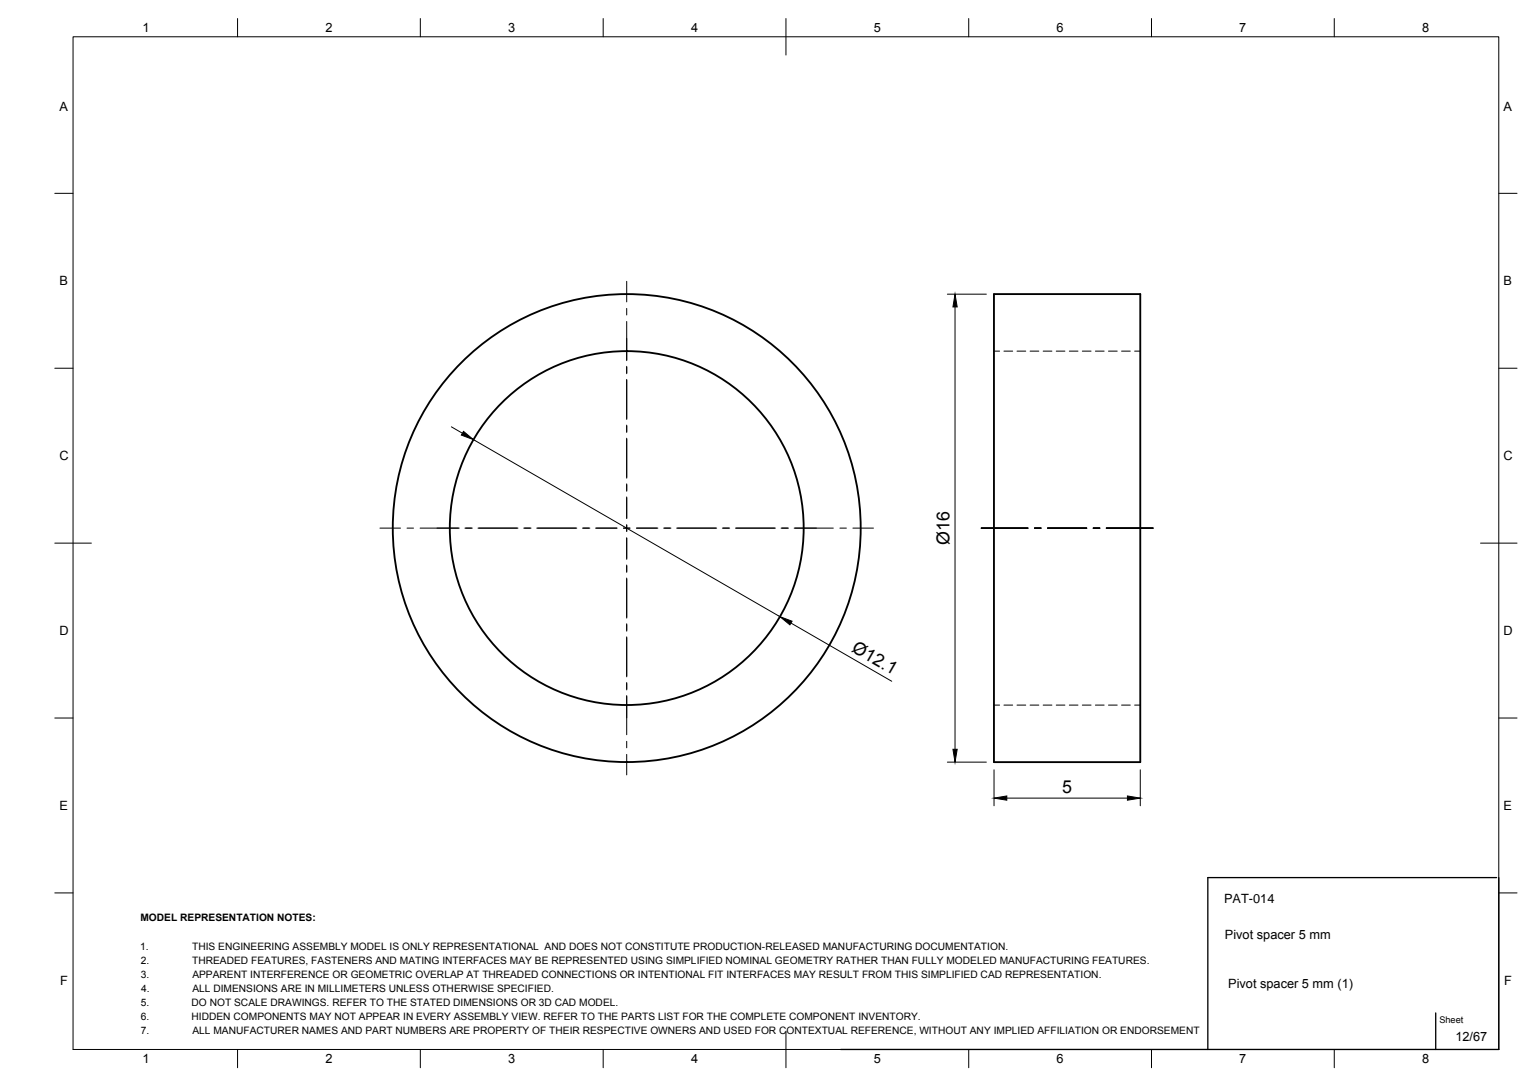
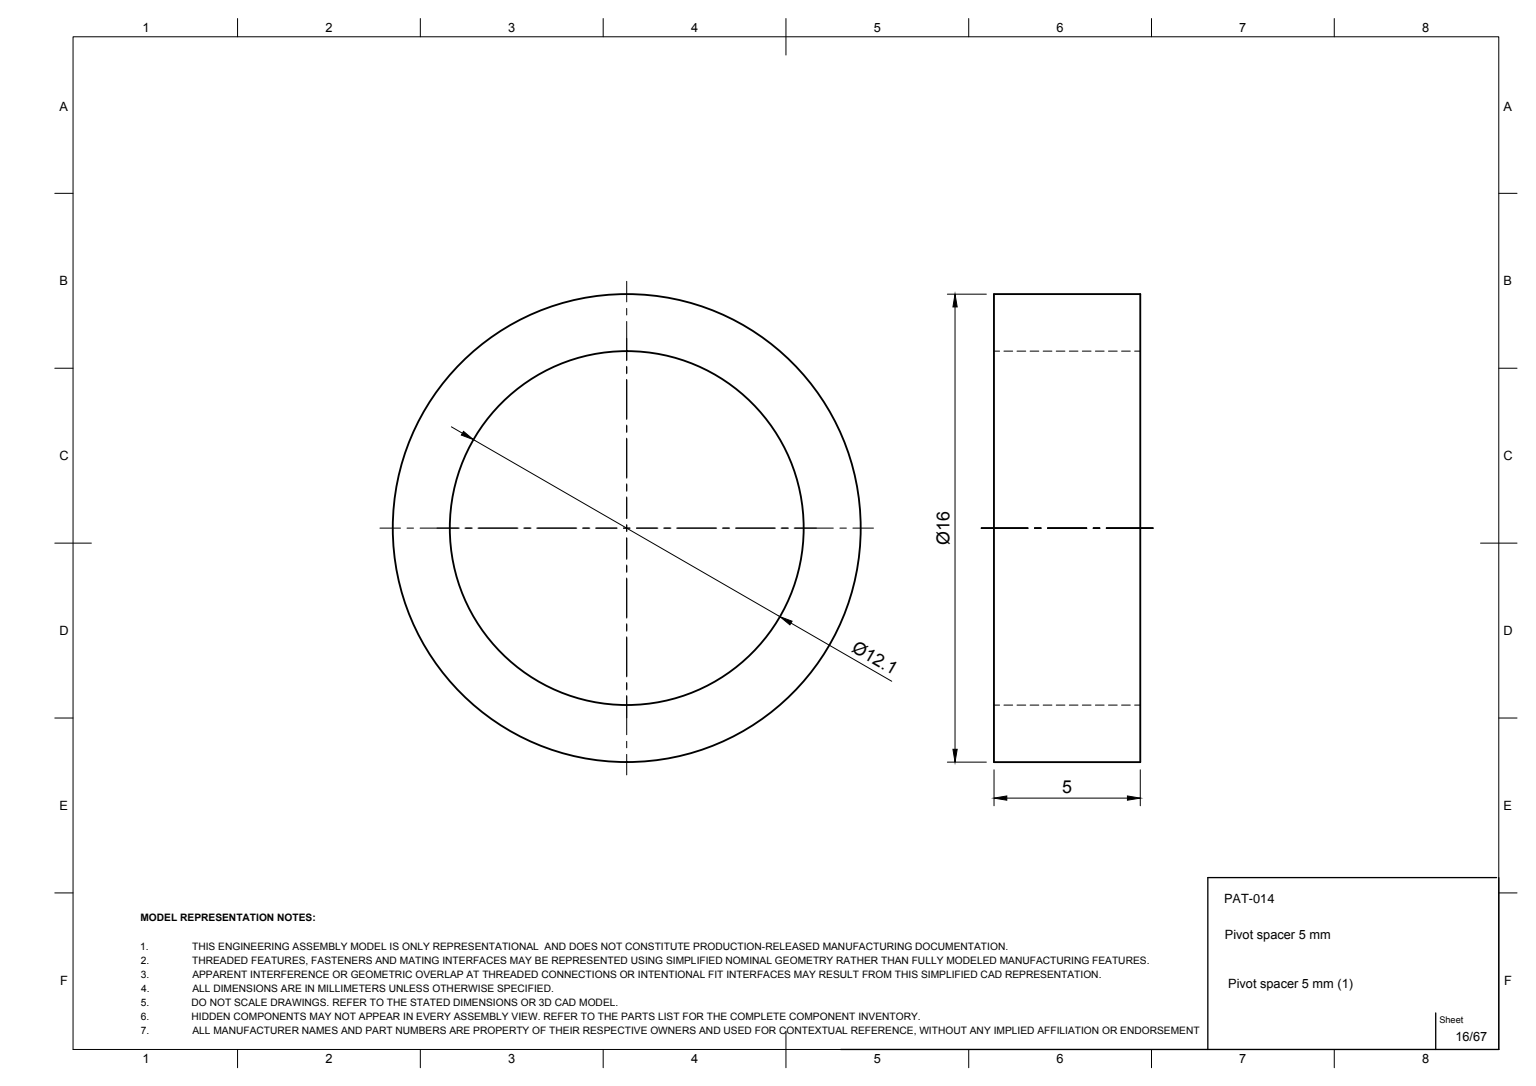
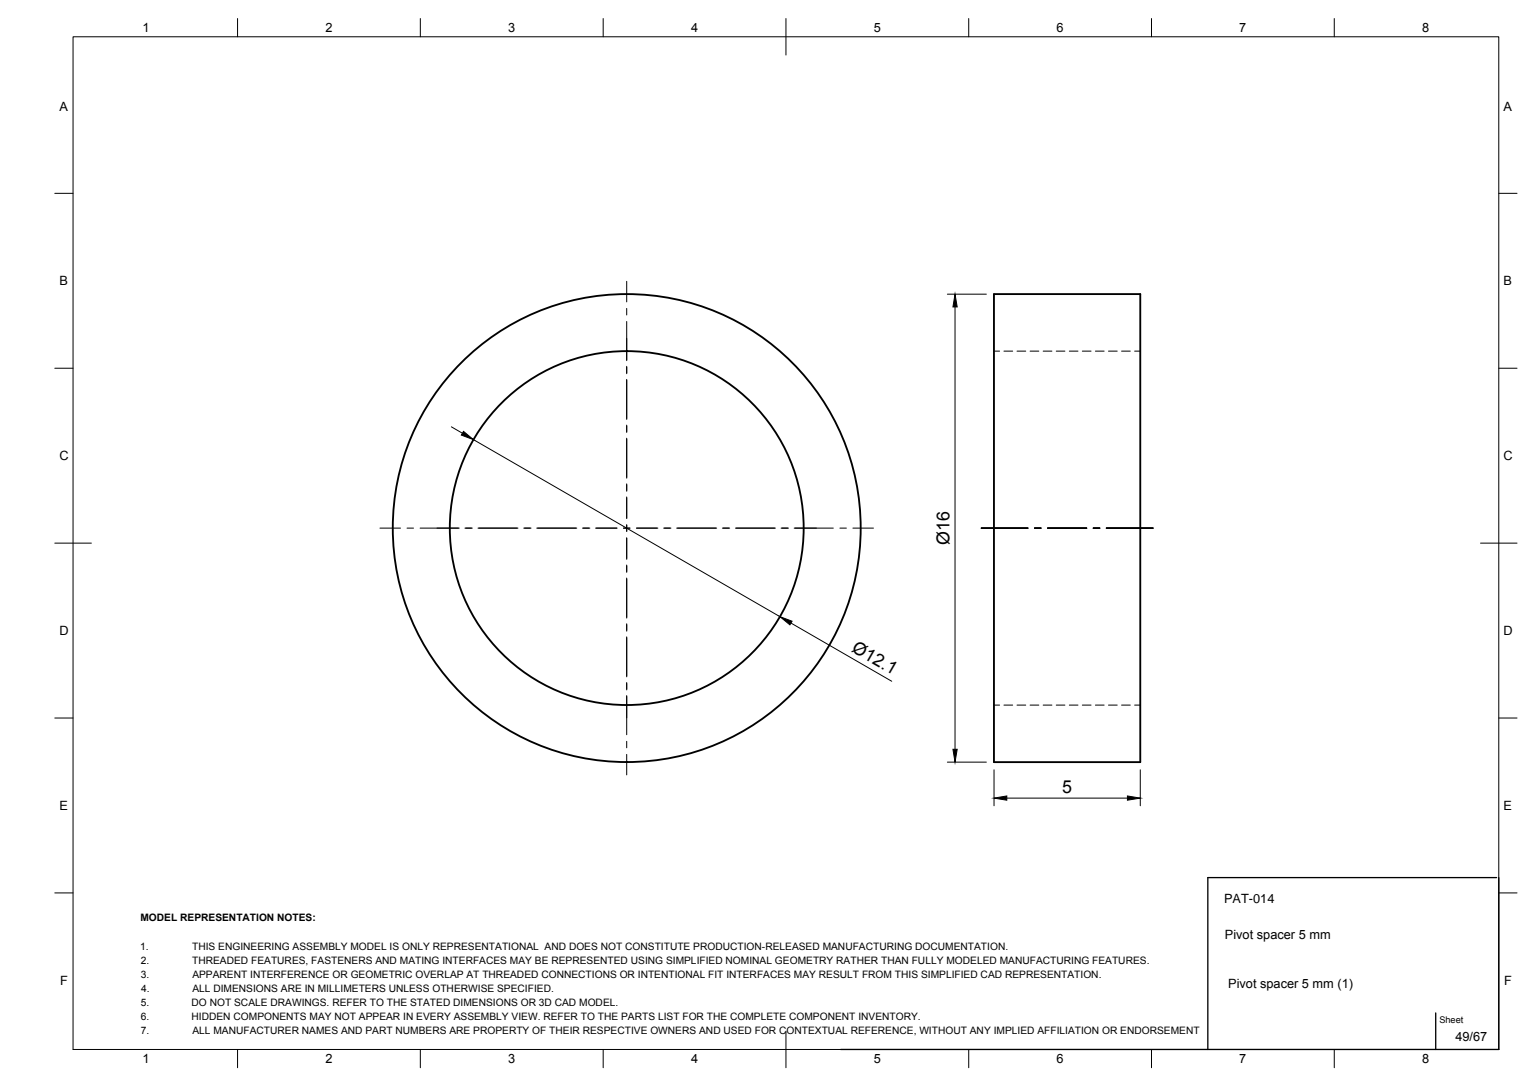
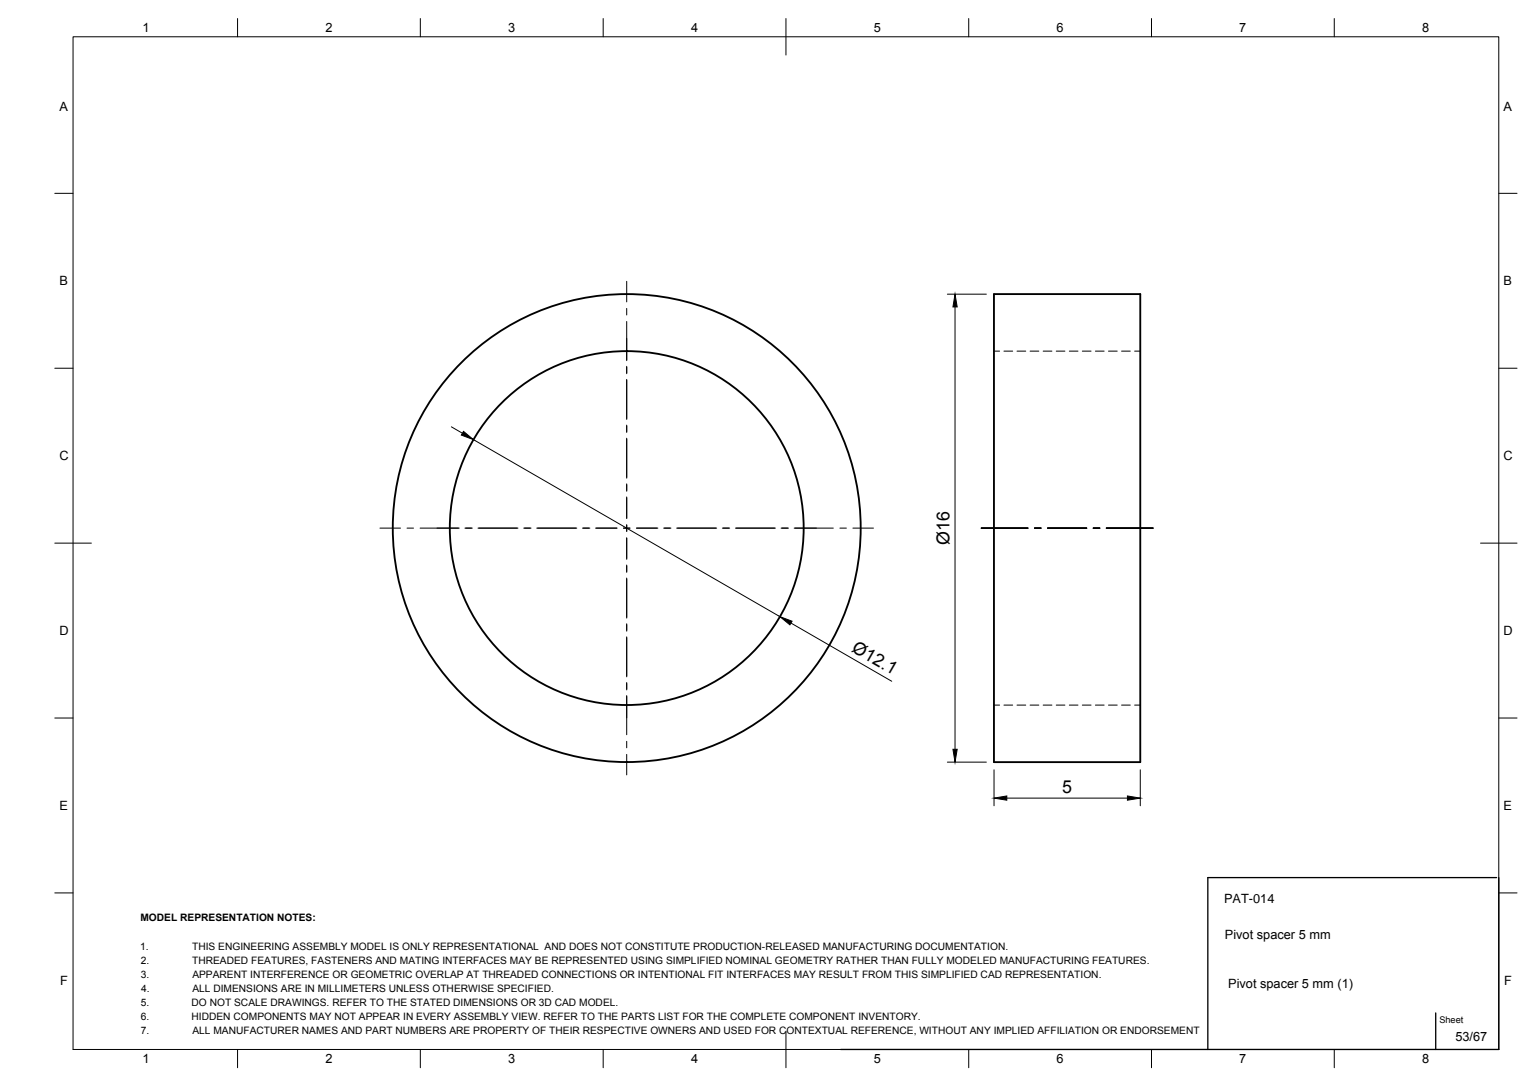
ISO-10303-21;
HEADER;
/* Generated by software containing ST-Developer
 * from STEP Tools, Inc. (www.steptools.com) 
 */

FILE_DESCRIPTION(
/* description */ ('Bin tilter linkage'),
/* implementation_level */ '2;1');

FILE_NAME(
/* name */ 'Pivot spacer 5 mm.step',
/* time_stamp */ '2026-10-28T03:26:24-07:00',
/* author */ (''),
/* organization */ (''),
/* preprocessor_version */ 'ST-DEVELOPER v20.2',
/* originating_system */ 'Autodesk Translation Framework v15.17.0.0',
/* authorisation */ '');

FILE_SCHEMA (('AUTOMOTIVE_DESIGN { 1 0 10303 214 3 1 1 }'));
ENDSEC;

DATA;
#10=MECHANICAL_DESIGN_GEOMETRIC_PRESENTATION_REPRESENTATION('',(#869),#23728);
#657=SHAPE_REPRESENTATION_RELATIONSHIP('SRR','None',#24121,#763);
#763=ADVANCED_BREP_SHAPE_REPRESENTATION('',(#983),#23621);
#869=STYLED_ITEM('',(#24779),#983);
#983=MANIFOLD_SOLID_BREP('Body1',#12399);
#1154=FACE_BOUND('',#2819,.T.);
#1155=FACE_BOUND('',#2821,.T.);
#1537=PLANE('',#13848);
#1538=PLANE('',#13849);
#1972=FACE_OUTER_BOUND('',#2816,.T.);
#1973=FACE_OUTER_BOUND('',#2817,.T.);
#1974=FACE_OUTER_BOUND('',#2818,.T.);
#1975=FACE_OUTER_BOUND('',#2820,.T.);
#2816=EDGE_LOOP('',(#8763,#8764,#8765,#8766));
#2817=EDGE_LOOP('',(#8767,#8768,#8769,#8770));
#2818=EDGE_LOOP('',(#8771));
#2819=EDGE_LOOP('',(#8772));
#2820=EDGE_LOOP('',(#8773));
#2821=EDGE_LOOP('',(#8774));
#3970=LINE('',#20166,#4645);
#3971=LINE('',#20172,#4646);
#4645=VECTOR('',#15931,0.605);
#4646=VECTOR('',#15938,0.8);
#5273=CIRCLE('',#13843,0.605);
#5274=CIRCLE('',#13844,0.605);
#5275=CIRCLE('',#13846,0.8);
#5276=CIRCLE('',#13847,0.8);
#6087=VERTEX_POINT('',#20163);
#6088=VERTEX_POINT('',#20165);
#6089=VERTEX_POINT('',#20169);
#6090=VERTEX_POINT('',#20171);
#7121=EDGE_CURVE('',#6087,#6087,#5273,.T.);
#7122=EDGE_CURVE('',#6087,#6088,#3970,.T.);
#7123=EDGE_CURVE('',#6088,#6088,#5274,.T.);
#7124=EDGE_CURVE('',#6089,#6089,#5275,.T.);
#7125=EDGE_CURVE('',#6089,#6090,#3971,.T.);
#7126=EDGE_CURVE('',#6090,#6090,#5276,.T.);
#8763=ORIENTED_EDGE('',*,*,#7121,.F.);
#8764=ORIENTED_EDGE('',*,*,#7122,.T.);
#8765=ORIENTED_EDGE('',*,*,#7123,.T.);
#8766=ORIENTED_EDGE('',*,*,#7122,.F.);
#8767=ORIENTED_EDGE('',*,*,#7124,.F.);
#8768=ORIENTED_EDGE('',*,*,#7125,.T.);
#8769=ORIENTED_EDGE('',*,*,#7126,.T.);
#8770=ORIENTED_EDGE('',*,*,#7125,.F.);
#8771=ORIENTED_EDGE('',*,*,#7124,.T.);
#8772=ORIENTED_EDGE('',*,*,#7121,.T.);
#8773=ORIENTED_EDGE('',*,*,#7126,.F.);
#8774=ORIENTED_EDGE('',*,*,#7123,.F.);
#11304=CYLINDRICAL_SURFACE('',#13842,0.605);
#11305=CYLINDRICAL_SURFACE('',#13845,0.8);
#11697=ADVANCED_FACE('',(#1972),#11304,.F.);
#11698=ADVANCED_FACE('',(#1973),#11305,.T.);
#11699=ADVANCED_FACE('',(#1974,#1154),#1537,.T.);
#11700=ADVANCED_FACE('',(#1975,#1155),#1538,.F.);
#12399=CLOSED_SHELL('',(#11697,#11698,#11699,#11700));
#13841=AXIS2_PLACEMENT_3D('',#20161,#15925,#15926);
#13842=AXIS2_PLACEMENT_3D('',#20162,#15927,#15928);
#13843=AXIS2_PLACEMENT_3D('',#20164,#15929,#15930);
#13844=AXIS2_PLACEMENT_3D('',#20167,#15932,#15933);
#13845=AXIS2_PLACEMENT_3D('',#20168,#15934,#15935);
#13846=AXIS2_PLACEMENT_3D('',#20170,#15936,#15937);
#13847=AXIS2_PLACEMENT_3D('',#20173,#15939,#15940);
#13848=AXIS2_PLACEMENT_3D('',#20174,#15941,#15942);
#13849=AXIS2_PLACEMENT_3D('',#20175,#15943,#15944);
#15925=DIRECTION('axis',(0.,0.,1.));
#15926=DIRECTION('refdir',(1.,0.,0.));
#15927=DIRECTION('center_axis',(0.,1.,0.));
#15928=DIRECTION('ref_axis',(1.,0.,0.));
#15929=DIRECTION('center_axis',(0.,-1.,0.));
#15930=DIRECTION('ref_axis',(1.,0.,0.));
#15931=DIRECTION('',(0.,-1.,0.));
#15932=DIRECTION('center_axis',(0.,-1.,0.));
#15933=DIRECTION('ref_axis',(1.,0.,0.));
#15934=DIRECTION('center_axis',(0.,1.,0.));
#15935=DIRECTION('ref_axis',(1.,0.,0.));
#15936=DIRECTION('center_axis',(0.,1.,0.));
#15937=DIRECTION('ref_axis',(1.,0.,0.));
#15938=DIRECTION('',(0.,-1.,0.));
#15939=DIRECTION('center_axis',(0.,1.,0.));
#15940=DIRECTION('ref_axis',(1.,0.,0.));
#15941=DIRECTION('center_axis',(0.,1.,0.));
#15942=DIRECTION('ref_axis',(1.,0.,0.));
#15943=DIRECTION('center_axis',(0.,1.,0.));
#15944=DIRECTION('ref_axis',(1.,0.,0.));
#20161=CARTESIAN_POINT('',(0.,0.,0.));
#20162=CARTESIAN_POINT('Origin',(0.,-1.,15.));
#20163=CARTESIAN_POINT('',(-0.605,-0.5,15.));
#20164=CARTESIAN_POINT('Origin',(0.,-0.5,15.));
#20165=CARTESIAN_POINT('',(-0.605,-1.,15.));
#20166=CARTESIAN_POINT('',(-0.605,-1.,15.));
#20167=CARTESIAN_POINT('Origin',(0.,-1.,15.));
#20168=CARTESIAN_POINT('Origin',(0.,-1.,15.));
#20169=CARTESIAN_POINT('',(-0.8,-0.5,15.));
#20170=CARTESIAN_POINT('Origin',(0.,-0.5,15.));
#20171=CARTESIAN_POINT('',(-0.8,-1.,15.));
#20172=CARTESIAN_POINT('',(-0.8,-1.,15.));
#20173=CARTESIAN_POINT('Origin',(0.,-1.,15.));
#20174=CARTESIAN_POINT('Origin',(0.,-0.5,15.));
#20175=CARTESIAN_POINT('Origin',(0.,-1.,15.));
#23504=UNCERTAINTY_MEASURE_WITH_UNIT(LENGTH_MEASURE(0.001),#23729,
'DISTANCE_ACCURACY_VALUE',
'Maximum model space distance between geometric entities at asserted c
onnectivities');
#23611=UNCERTAINTY_MEASURE_WITH_UNIT(LENGTH_MEASURE(0.001),#23729,
'DISTANCE_ACCURACY_VALUE',
'Maximum model space distance between geometric entities at asserted c
onnectivities');
#23621=(
GEOMETRIC_REPRESENTATION_CONTEXT(3)
GLOBAL_UNCERTAINTY_ASSIGNED_CONTEXT((#23504))
GLOBAL_UNIT_ASSIGNED_CONTEXT((#23729,#23731,#23732))
REPRESENTATION_CONTEXT('','3D')
);
#23728=(
GEOMETRIC_REPRESENTATION_CONTEXT(3)
GLOBAL_UNCERTAINTY_ASSIGNED_CONTEXT((#23611))
GLOBAL_UNIT_ASSIGNED_CONTEXT((#23729,#23731,#23732))
REPRESENTATION_CONTEXT('','3D')
);
#23729=(
LENGTH_UNIT()
NAMED_UNIT(*)
SI_UNIT(.CENTI.,.METRE.)
);
#23731=(
NAMED_UNIT(*)
PLANE_ANGLE_UNIT()
SI_UNIT($,.RADIAN.)
);
#23732=(
NAMED_UNIT(*)
SI_UNIT($,.STERADIAN.)
SOLID_ANGLE_UNIT()
);
#23742=SHAPE_DEFINITION_REPRESENTATION(#23858,#24121);
#23858=PRODUCT_DEFINITION_SHAPE('',$,#24238);
#24121=SHAPE_REPRESENTATION('',(#13841),#23621);
#24228=PRODUCT_DEFINITION_CONTEXT('part definition',#24578,'design');
#24238=PRODUCT_DEFINITION('Pivot spacer 5 mm','Pivot spacer 5 mm',#24354,
#24228);
#24354=PRODUCT_DEFINITION_FORMATION('',$,#24589);
#24578=APPLICATION_CONTEXT(
'Core Data for Automotive Mechanical Design Process');
#24579=PRODUCT_CONTEXT('part definition',#24578,'mechanical');
#24589=PRODUCT('Pivot spacer 5 mm','Pivot spacer 5 mm',
'Pivot spacer 5 mm',(#24579));
#24773=COLOUR_RGB('Off White',0.89,0.88,0.83);
#24774=FILL_AREA_STYLE_COLOUR('',#24773);
#24775=FILL_AREA_STYLE('',(#24774));
#24776=SURFACE_STYLE_FILL_AREA(#24775);
#24777=SURFACE_SIDE_STYLE('',(#24776));
#24778=SURFACE_STYLE_USAGE(.BOTH.,#24777);
#24779=PRESENTATION_STYLE_ASSIGNMENT((#24778));
ENDSEC;
END-ISO-10303-21;
